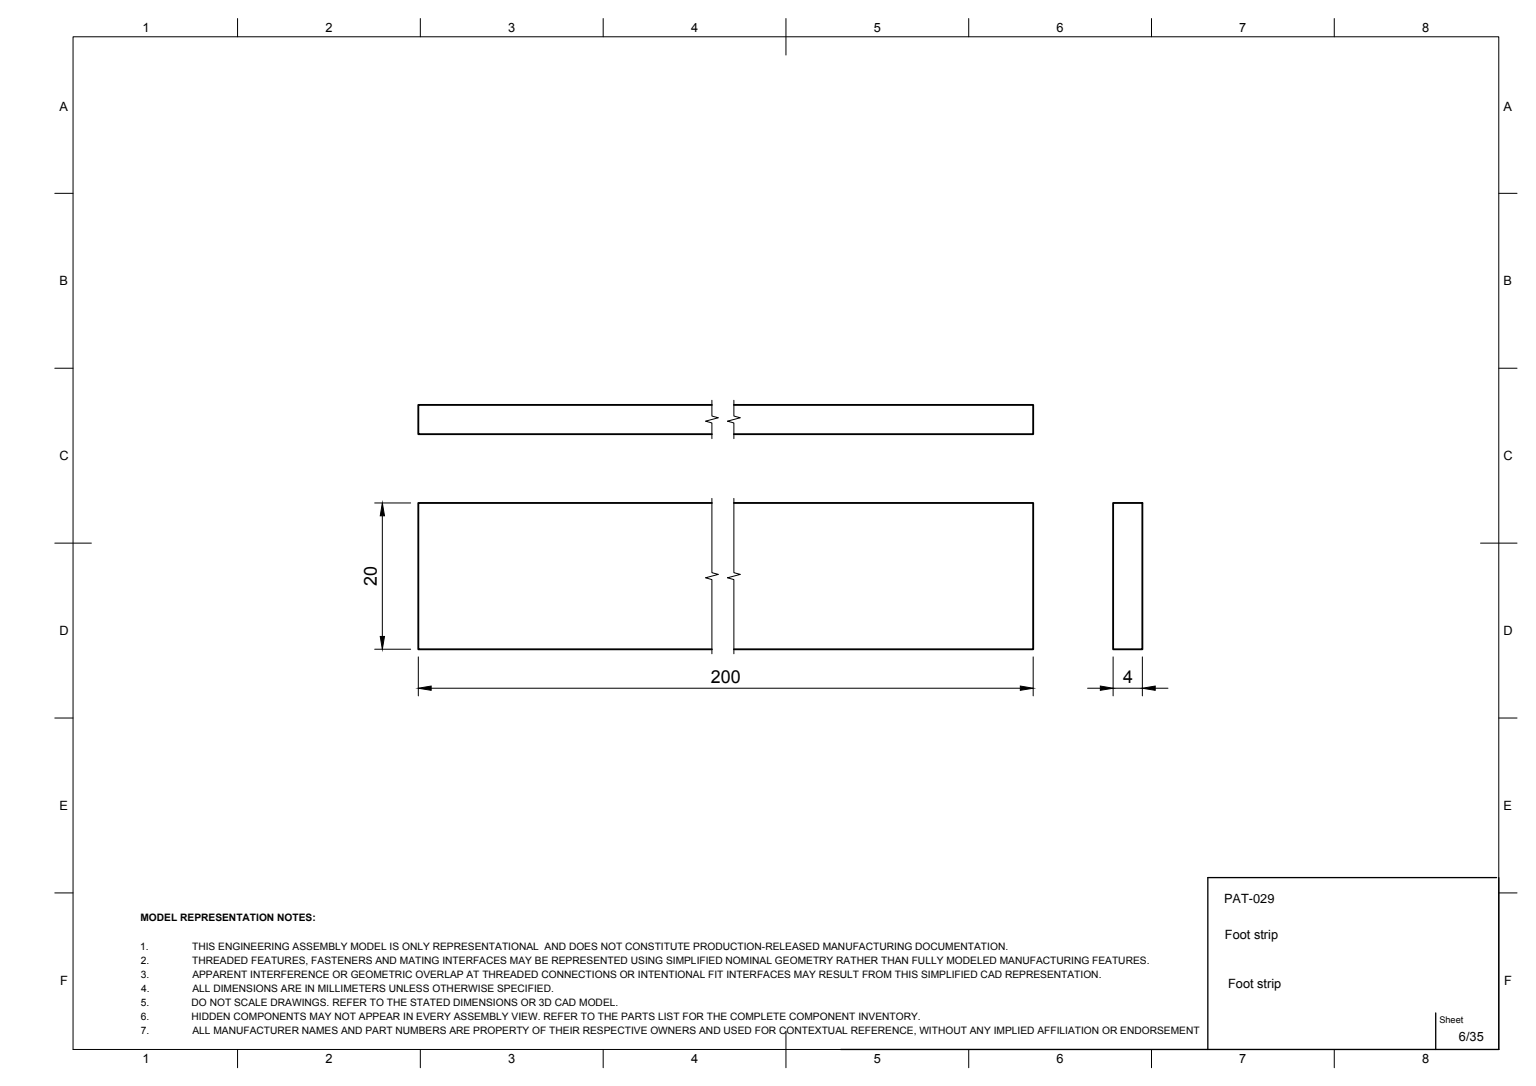
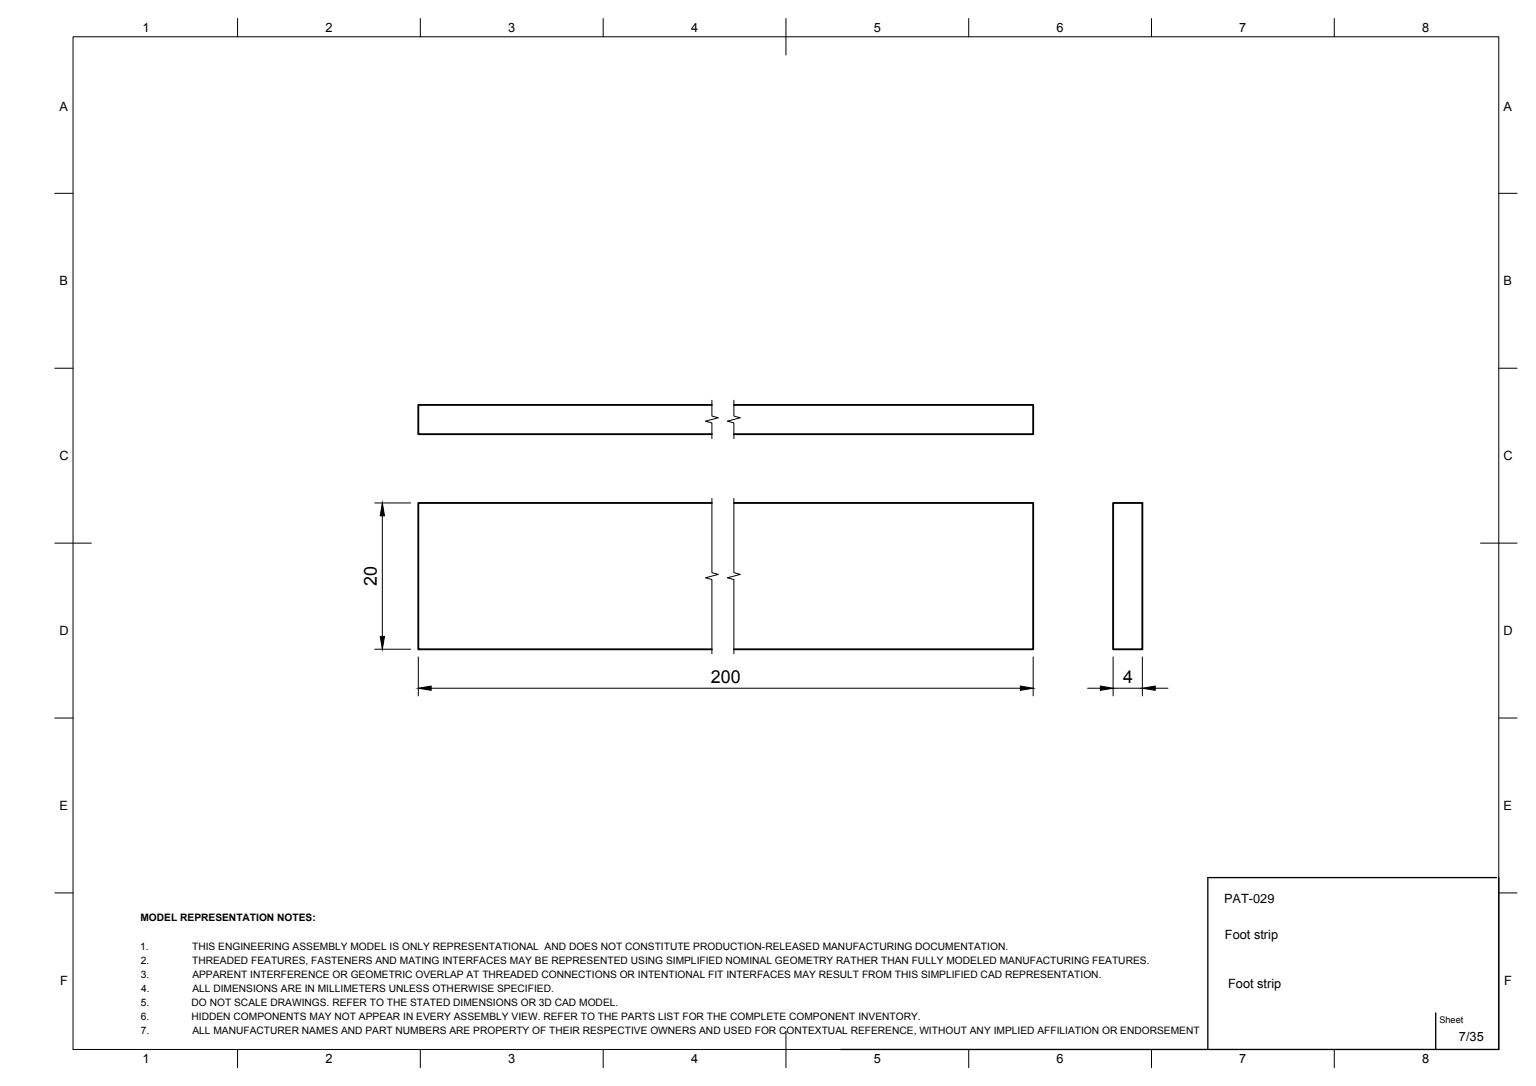
ISO-10303-21;
HEADER;
/* Generated by software containing ST-Developer
 * from STEP Tools, Inc. (www.steptools.com) 
 */

FILE_DESCRIPTION(
/* description */ ('Door-style hinge test fixture with detent'),
/* implementation_level */ '2;1');

FILE_NAME(
/* name */ 'Foot strip.step',
/* time_stamp */ '2026-10-28T03:24:57-07:00',
/* author */ (''),
/* organization */ (''),
/* preprocessor_version */ 'ST-DEVELOPER v20.2',
/* originating_system */ 'Autodesk Translation Framework v15.17.0.0',
/* authorisation */ '');

FILE_SCHEMA (('AUTOMOTIVE_DESIGN { 1 0 10303 214 3 1 1 }'));
ENDSEC;

DATA;
#10=MECHANICAL_DESIGN_GEOMETRIC_PRESENTATION_REPRESENTATION('',(#323),#9813);
#261=SHAPE_REPRESENTATION_RELATIONSHIP('SRR','None',#9938,#292);
#292=ADVANCED_BREP_SHAPE_REPRESENTATION('',(#363),#9781);
#323=STYLED_ITEM('',(#10169),#363);
#363=MANIFOLD_SOLID_BREP('Body1',#4754);
#506=PLANE('',#5160);
#507=PLANE('',#5161);
#508=PLANE('',#5162);
#509=PLANE('',#5163);
#510=PLANE('',#5164);
#511=PLANE('',#5165);
#673=FACE_OUTER_BOUND('',#966,.T.);
#674=FACE_OUTER_BOUND('',#967,.T.);
#675=FACE_OUTER_BOUND('',#968,.T.);
#676=FACE_OUTER_BOUND('',#969,.T.);
#677=FACE_OUTER_BOUND('',#970,.T.);
#678=FACE_OUTER_BOUND('',#971,.T.);
#966=EDGE_LOOP('',(#3255,#3256,#3257,#3258));
#967=EDGE_LOOP('',(#3259,#3260,#3261,#3262));
#968=EDGE_LOOP('',(#3263,#3264,#3265,#3266));
#969=EDGE_LOOP('',(#3267,#3268,#3269,#3270));
#970=EDGE_LOOP('',(#3271,#3272,#3273,#3274));
#971=EDGE_LOOP('',(#3275,#3276,#3277,#3278));
#1350=LINE('',#7354,#1670);
#1351=LINE('',#7356,#1671);
#1352=LINE('',#7358,#1672);
#1353=LINE('',#7359,#1673);
#1354=LINE('',#7362,#1674);
#1355=LINE('',#7364,#1675);
#1356=LINE('',#7365,#1676);
#1357=LINE('',#7368,#1677);
#1358=LINE('',#7370,#1678);
#1359=LINE('',#7371,#1679);
#1360=LINE('',#7373,#1680);
#1361=LINE('',#7374,#1681);
#1670=VECTOR('',#5813,1.);
#1671=VECTOR('',#5814,1.);
#1672=VECTOR('',#5815,1.);
#1673=VECTOR('',#5816,1.);
#1674=VECTOR('',#5819,1.);
#1675=VECTOR('',#5820,1.);
#1676=VECTOR('',#5821,1.);
#1677=VECTOR('',#5824,1.);
#1678=VECTOR('',#5825,1.);
#1679=VECTOR('',#5826,1.);
#1680=VECTOR('',#5829,1.);
#1681=VECTOR('',#5830,1.);
#2237=VERTEX_POINT('',#7352);
#2238=VERTEX_POINT('',#7353);
#2239=VERTEX_POINT('',#7355);
#2240=VERTEX_POINT('',#7357);
#2241=VERTEX_POINT('',#7361);
#2242=VERTEX_POINT('',#7363);
#2243=VERTEX_POINT('',#7367);
#2244=VERTEX_POINT('',#7369);
#2644=EDGE_CURVE('',#2237,#2238,#1350,.T.);
#2645=EDGE_CURVE('',#2238,#2239,#1351,.T.);
#2646=EDGE_CURVE('',#2240,#2239,#1352,.T.);
#2647=EDGE_CURVE('',#2237,#2240,#1353,.T.);
#2648=EDGE_CURVE('',#2241,#2237,#1354,.T.);
#2649=EDGE_CURVE('',#2242,#2240,#1355,.T.);
#2650=EDGE_CURVE('',#2241,#2242,#1356,.T.);
#2651=EDGE_CURVE('',#2243,#2241,#1357,.T.);
#2652=EDGE_CURVE('',#2244,#2242,#1358,.T.);
#2653=EDGE_CURVE('',#2243,#2244,#1359,.T.);
#2654=EDGE_CURVE('',#2238,#2243,#1360,.T.);
#2655=EDGE_CURVE('',#2239,#2244,#1361,.T.);
#3255=ORIENTED_EDGE('',*,*,#2644,.T.);
#3256=ORIENTED_EDGE('',*,*,#2645,.T.);
#3257=ORIENTED_EDGE('',*,*,#2646,.F.);
#3258=ORIENTED_EDGE('',*,*,#2647,.F.);
#3259=ORIENTED_EDGE('',*,*,#2648,.T.);
#3260=ORIENTED_EDGE('',*,*,#2647,.T.);
#3261=ORIENTED_EDGE('',*,*,#2649,.F.);
#3262=ORIENTED_EDGE('',*,*,#2650,.F.);
#3263=ORIENTED_EDGE('',*,*,#2651,.T.);
#3264=ORIENTED_EDGE('',*,*,#2650,.T.);
#3265=ORIENTED_EDGE('',*,*,#2652,.F.);
#3266=ORIENTED_EDGE('',*,*,#2653,.F.);
#3267=ORIENTED_EDGE('',*,*,#2654,.T.);
#3268=ORIENTED_EDGE('',*,*,#2653,.T.);
#3269=ORIENTED_EDGE('',*,*,#2655,.F.);
#3270=ORIENTED_EDGE('',*,*,#2645,.F.);
#3271=ORIENTED_EDGE('',*,*,#2655,.T.);
#3272=ORIENTED_EDGE('',*,*,#2652,.T.);
#3273=ORIENTED_EDGE('',*,*,#2649,.T.);
#3274=ORIENTED_EDGE('',*,*,#2646,.T.);
#3275=ORIENTED_EDGE('',*,*,#2654,.F.);
#3276=ORIENTED_EDGE('',*,*,#2644,.F.);
#3277=ORIENTED_EDGE('',*,*,#2648,.F.);
#3278=ORIENTED_EDGE('',*,*,#2651,.F.);
#4478=ADVANCED_FACE('',(#673),#506,.T.);
#4479=ADVANCED_FACE('',(#674),#507,.T.);
#4480=ADVANCED_FACE('',(#675),#508,.T.);
#4481=ADVANCED_FACE('',(#676),#509,.T.);
#4482=ADVANCED_FACE('',(#677),#510,.T.);
#4483=ADVANCED_FACE('',(#678),#511,.F.);
#4754=CLOSED_SHELL('',(#4478,#4479,#4480,#4481,#4482,#4483));
#5159=AXIS2_PLACEMENT_3D('',#7350,#5809,#5810);
#5160=AXIS2_PLACEMENT_3D('',#7351,#5811,#5812);
#5161=AXIS2_PLACEMENT_3D('',#7360,#5817,#5818);
#5162=AXIS2_PLACEMENT_3D('',#7366,#5822,#5823);
#5163=AXIS2_PLACEMENT_3D('',#7372,#5827,#5828);
#5164=AXIS2_PLACEMENT_3D('',#7375,#5831,#5832);
#5165=AXIS2_PLACEMENT_3D('',#7376,#5833,#5834);
#5809=DIRECTION('axis',(0.,0.,1.));
#5810=DIRECTION('refdir',(1.,0.,0.));
#5811=DIRECTION('center_axis',(0.,1.,0.));
#5812=DIRECTION('ref_axis',(-1.,0.,0.));
#5813=DIRECTION('',(-1.,0.,0.));
#5814=DIRECTION('',(0.,0.,1.));
#5815=DIRECTION('',(-1.,0.,0.));
#5816=DIRECTION('',(0.,0.,1.));
#5817=DIRECTION('center_axis',(1.,0.,0.));
#5818=DIRECTION('ref_axis',(0.,1.,0.));
#5819=DIRECTION('',(0.,1.,0.));
#5820=DIRECTION('',(0.,1.,0.));
#5821=DIRECTION('',(0.,0.,1.));
#5822=DIRECTION('center_axis',(0.,-1.,0.));
#5823=DIRECTION('ref_axis',(1.,0.,0.));
#5824=DIRECTION('',(1.,0.,0.));
#5825=DIRECTION('',(1.,0.,0.));
#5826=DIRECTION('',(0.,0.,1.));
#5827=DIRECTION('center_axis',(-1.,0.,0.));
#5828=DIRECTION('ref_axis',(0.,-1.,0.));
#5829=DIRECTION('',(0.,-1.,0.));
#5830=DIRECTION('',(0.,-1.,0.));
#5831=DIRECTION('center_axis',(0.,0.,1.));
#5832=DIRECTION('ref_axis',(1.,0.,0.));
#5833=DIRECTION('center_axis',(0.,0.,1.));
#5834=DIRECTION('ref_axis',(1.,0.,0.));
#7350=CARTESIAN_POINT('',(0.,0.,0.));
#7351=CARTESIAN_POINT('Origin',(-11.5,13.5,-1.4));
#7352=CARTESIAN_POINT('',(-11.5,13.5,-1.4));
#7353=CARTESIAN_POINT('',(-13.5,13.5,-1.4));
#7354=CARTESIAN_POINT('',(-11.5,13.5,-1.4));
#7355=CARTESIAN_POINT('',(-13.5,13.5,-1.));
#7356=CARTESIAN_POINT('',(-13.5,13.5,-1.4));
#7357=CARTESIAN_POINT('',(-11.5,13.5,-1.));
#7358=CARTESIAN_POINT('',(-11.5,13.5,-1.));
#7359=CARTESIAN_POINT('',(-11.5,13.5,-1.4));
#7360=CARTESIAN_POINT('Origin',(-11.5,-6.5,-1.4));
#7361=CARTESIAN_POINT('',(-11.5,-6.5,-1.4));
#7362=CARTESIAN_POINT('',(-11.5,-6.5,-1.4));
#7363=CARTESIAN_POINT('',(-11.5,-6.5,-1.));
#7364=CARTESIAN_POINT('',(-11.5,-6.5,-1.));
#7365=CARTESIAN_POINT('',(-11.5,-6.5,-1.4));
#7366=CARTESIAN_POINT('Origin',(-13.5,-6.5,-1.4));
#7367=CARTESIAN_POINT('',(-13.5,-6.5,-1.4));
#7368=CARTESIAN_POINT('',(-13.5,-6.5,-1.4));
#7369=CARTESIAN_POINT('',(-13.5,-6.5,-1.));
#7370=CARTESIAN_POINT('',(-13.5,-6.5,-1.));
#7371=CARTESIAN_POINT('',(-13.5,-6.5,-1.4));
#7372=CARTESIAN_POINT('Origin',(-13.5,13.5,-1.4));
#7373=CARTESIAN_POINT('',(-13.5,13.5,-1.4));
#7374=CARTESIAN_POINT('',(-13.5,13.5,-1.));
#7375=CARTESIAN_POINT('Origin',(-12.5,3.5,-1.));
#7376=CARTESIAN_POINT('Origin',(-12.5,3.5,-1.4));
#9745=UNCERTAINTY_MEASURE_WITH_UNIT(LENGTH_MEASURE(0.001),#9814,
'DISTANCE_ACCURACY_VALUE',
'Maximum model space distance between geometric entities at asserted c
onnectivities');
#9777=UNCERTAINTY_MEASURE_WITH_UNIT(LENGTH_MEASURE(0.001),#9814,
'DISTANCE_ACCURACY_VALUE',
'Maximum model space distance between geometric entities at asserted c
onnectivities');
#9781=(
GEOMETRIC_REPRESENTATION_CONTEXT(3)
GLOBAL_UNCERTAINTY_ASSIGNED_CONTEXT((#9745))
GLOBAL_UNIT_ASSIGNED_CONTEXT((#9814,#9816,#9817))
REPRESENTATION_CONTEXT('','3D')
);
#9813=(
GEOMETRIC_REPRESENTATION_CONTEXT(3)
GLOBAL_UNCERTAINTY_ASSIGNED_CONTEXT((#9777))
GLOBAL_UNIT_ASSIGNED_CONTEXT((#9814,#9816,#9817))
REPRESENTATION_CONTEXT('','3D')
);
#9814=(
LENGTH_UNIT()
NAMED_UNIT(*)
SI_UNIT(.CENTI.,.METRE.)
);
#9816=(
NAMED_UNIT(*)
PLANE_ANGLE_UNIT()
SI_UNIT($,.RADIAN.)
);
#9817=(
NAMED_UNIT(*)
SI_UNIT($,.STERADIAN.)
SOLID_ANGLE_UNIT()
);
#9821=SHAPE_DEFINITION_REPRESENTATION(#9856,#9938);
#9856=PRODUCT_DEFINITION_SHAPE('',$,#9974);
#9938=SHAPE_REPRESENTATION('',(#5159),#9781);
#9970=PRODUCT_DEFINITION_CONTEXT('part definition',#10077,'design');
#9974=PRODUCT_DEFINITION('Foot strip','Foot strip',#10009,#9970);
#10009=PRODUCT_DEFINITION_FORMATION('',$,#10082);
#10077=APPLICATION_CONTEXT(
'Core Data for Automotive Mechanical Design Process');
#10078=PRODUCT_CONTEXT('part definition',#10077,'mechanical');
#10082=PRODUCT('Foot strip','Foot strip','Foot strip',(#10078));
#10163=COLOUR_RGB('Light Blue',0.38,0.62,0.78);
#10164=FILL_AREA_STYLE_COLOUR('',#10163);
#10165=FILL_AREA_STYLE('',(#10164));
#10166=SURFACE_STYLE_FILL_AREA(#10165);
#10167=SURFACE_SIDE_STYLE('',(#10166));
#10168=SURFACE_STYLE_USAGE(.BOTH.,#10167);
#10169=PRESENTATION_STYLE_ASSIGNMENT((#10168));
ENDSEC;
END-ISO-10303-21;
